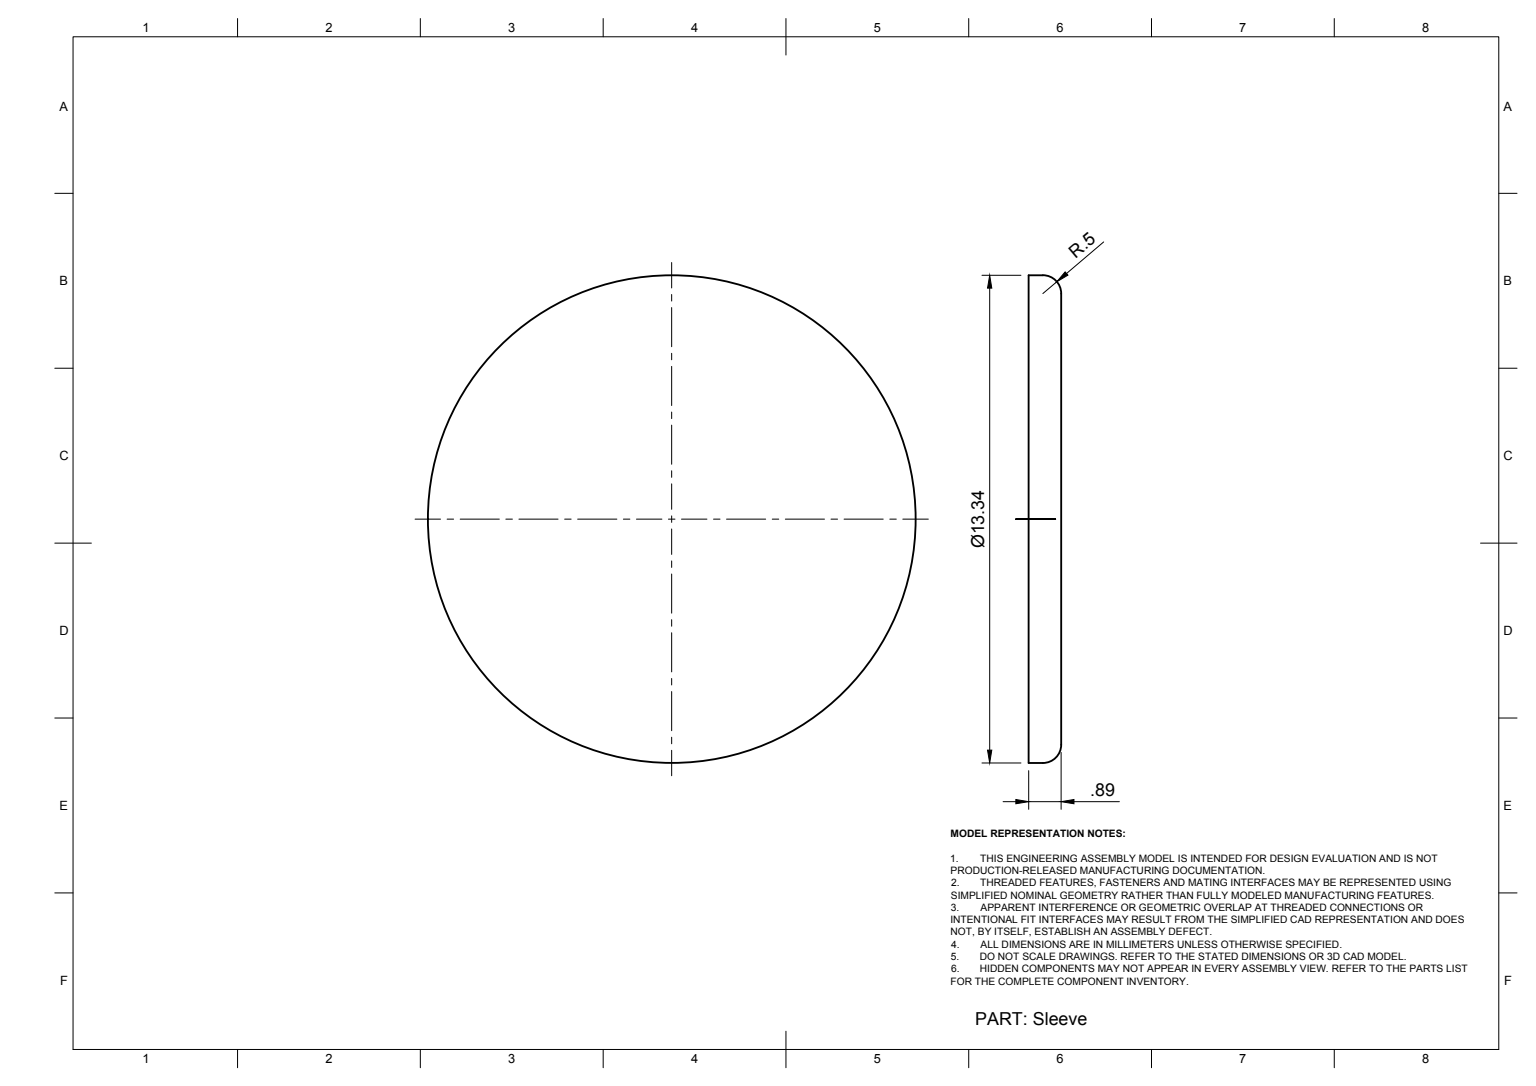
ISO-10303-21;
HEADER;
/* Generated by software containing ST-Developer
 * from STEP Tools, Inc. (www.steptools.com) 
 */

FILE_DESCRIPTION(
/* description */ (''),
/* implementation_level */ '2;1');

FILE_NAME(
/* name */ 'Sleeve.step',
/* time_stamp */ '2026-10-05T01:33:24-07:00',
/* author */ (''),
/* organization */ (''),
/* preprocessor_version */ 'ST-DEVELOPER v20.2',
/* originating_system */ 'Autodesk Translation Framework v15.15.0.0',
/* authorisation */ '');

FILE_SCHEMA (('AUTOMOTIVE_DESIGN { 1 0 10303 214 3 1 1 }'));
ENDSEC;

DATA;
#10=MECHANICAL_DESIGN_GEOMETRIC_PRESENTATION_REPRESENTATION('',(#89),#1128);
#54=TOROIDAL_SURFACE('',#709,6.1693331034204,0.499999999999997);
#69=SHAPE_REPRESENTATION_RELATIONSHIP('SRR','None',#1173,#79);
#79=ADVANCED_BREP_SHAPE_REPRESENTATION('',(#99),#1125);
#89=STYLED_ITEM('',(#1227),#99);
#99=MANIFOLD_SOLID_BREP('Body1',#528);
#114=LINE('',#1064,#131);
#131=VECTOR('',#895,6.66933310342039);
#143=CYLINDRICAL_SURFACE('',#712,6.66933310342039);
#175=FACE_OUTER_BOUND('',#216,.T.);
#176=FACE_OUTER_BOUND('',#217,.T.);
#177=FACE_OUTER_BOUND('',#218,.T.);
#178=FACE_OUTER_BOUND('',#219,.T.);
#216=EDGE_LOOP('',(#426));
#217=EDGE_LOOP('',(#427));
#218=EDGE_LOOP('',(#428,#429,#430,#431));
#219=EDGE_LOOP('',(#432,#433,#434,#435));
#253=CIRCLE('',#706,6.66933310342039);
#254=CIRCLE('',#708,6.16933310342039);
#255=CIRCLE('',#710,6.66933310342039);
#256=CIRCLE('',#711,0.499999999999997);
#287=VERTEX_POINT('',#1054);
#288=VERTEX_POINT('',#1057);
#289=VERTEX_POINT('',#1060);
#335=EDGE_CURVE('',#287,#287,#253,.T.);
#336=EDGE_CURVE('',#288,#288,#254,.T.);
#337=EDGE_CURVE('',#289,#289,#255,.T.);
#338=EDGE_CURVE('',#289,#288,#256,.T.);
#339=EDGE_CURVE('',#287,#289,#114,.T.);
#426=ORIENTED_EDGE('',*,*,#335,.T.);
#427=ORIENTED_EDGE('',*,*,#336,.F.);
#428=ORIENTED_EDGE('',*,*,#337,.F.);
#429=ORIENTED_EDGE('',*,*,#338,.T.);
#430=ORIENTED_EDGE('',*,*,#336,.T.);
#431=ORIENTED_EDGE('',*,*,#338,.F.);
#432=ORIENTED_EDGE('',*,*,#335,.F.);
#433=ORIENTED_EDGE('',*,*,#339,.T.);
#434=ORIENTED_EDGE('',*,*,#337,.T.);
#435=ORIENTED_EDGE('',*,*,#339,.F.);
#474=PLANE('',#705);
#475=PLANE('',#707);
#509=ADVANCED_FACE('',(#175),#474,.T.);
#510=ADVANCED_FACE('',(#176),#475,.T.);
#511=ADVANCED_FACE('',(#177),#54,.T.);
#512=ADVANCED_FACE('',(#178),#143,.T.);
#528=CLOSED_SHELL('',(#509,#510,#511,#512));
#704=AXIS2_PLACEMENT_3D('',#1052,#877,#878);
#705=AXIS2_PLACEMENT_3D('',#1053,#879,#880);
#706=AXIS2_PLACEMENT_3D('',#1055,#881,#882);
#707=AXIS2_PLACEMENT_3D('',#1056,#883,#884);
#708=AXIS2_PLACEMENT_3D('',#1058,#885,#886);
#709=AXIS2_PLACEMENT_3D('',#1059,#887,#888);
#710=AXIS2_PLACEMENT_3D('',#1061,#889,#890);
#711=AXIS2_PLACEMENT_3D('',#1062,#891,#892);
#712=AXIS2_PLACEMENT_3D('',#1063,#893,#894);
#877=DIRECTION('axis',(0.,0.,1.));
#878=DIRECTION('refdir',(1.,0.,0.));
#879=DIRECTION('center_axis',(1.,0.,0.));
#880=DIRECTION('ref_axis',(0.,0.,-1.));
#881=DIRECTION('center_axis',(1.,0.,0.));
#882=DIRECTION('ref_axis',(0.,0.,-1.));
#883=DIRECTION('center_axis',(-1.,0.,0.));
#884=DIRECTION('ref_axis',(0.,0.,1.));
#885=DIRECTION('center_axis',(1.,0.,0.));
#886=DIRECTION('ref_axis',(0.,0.,-1.));
#887=DIRECTION('center_axis',(1.,0.,0.));
#888=DIRECTION('ref_axis',(0.,0.,-1.));
#889=DIRECTION('center_axis',(1.,0.,0.));
#890=DIRECTION('ref_axis',(0.,0.,-1.));
#891=DIRECTION('center_axis',(0.,-1.,-1.22464679914735E-16));
#892=DIRECTION('ref_axis',(0.,-1.22464679914735E-16,1.));
#893=DIRECTION('center_axis',(1.,0.,0.));
#894=DIRECTION('ref_axis',(0.,0.,-1.));
#895=DIRECTION('',(-1.,0.,0.));
#1052=CARTESIAN_POINT('',(0.,0.,0.));
#1053=CARTESIAN_POINT('Origin',(31.9264360344922,0.,0.));
#1054=CARTESIAN_POINT('',(31.9264360344922,-8.16757743755127E-16,6.66933310342039));
#1055=CARTESIAN_POINT('Origin',(31.9264360344922,0.,0.));
#1056=CARTESIAN_POINT('Origin',(31.0379185953459,0.,-6.16933310342039));
#1057=CARTESIAN_POINT('',(31.0379185953459,-7.55525403797759E-16,6.16933310342039));
#1058=CARTESIAN_POINT('Origin',(31.0379185953459,0.,0.));
#1059=CARTESIAN_POINT('Origin',(31.5379185953459,0.,0.));
#1060=CARTESIAN_POINT('',(31.5379185953459,-8.16757743755127E-16,6.66933310342039));
#1061=CARTESIAN_POINT('Origin',(31.5379185953459,0.,0.));
#1062=CARTESIAN_POINT('Origin',(31.5379185953459,-7.5552540379776E-16,6.1693331034204));
#1063=CARTESIAN_POINT('Origin',(31.7321773149191,0.,0.));
#1064=CARTESIAN_POINT('',(31.7321773149191,-8.16757743755127E-16,6.66933310342039));
#1113=UNCERTAINTY_MEASURE_WITH_UNIT(LENGTH_MEASURE(0.01),#1129,
'DISTANCE_ACCURACY_VALUE',
'Maximum model space distance between geometric entities at asserted c
onnectivities');
#1116=UNCERTAINTY_MEASURE_WITH_UNIT(LENGTH_MEASURE(0.01),#1129,
'DISTANCE_ACCURACY_VALUE',
'Maximum model space distance between geometric entities at asserted c
onnectivities');
#1125=(
GEOMETRIC_REPRESENTATION_CONTEXT(3)
GLOBAL_UNCERTAINTY_ASSIGNED_CONTEXT((#1113))
GLOBAL_UNIT_ASSIGNED_CONTEXT((#1129,#1131,#1132))
REPRESENTATION_CONTEXT('','3D')
);
#1128=(
GEOMETRIC_REPRESENTATION_CONTEXT(3)
GLOBAL_UNCERTAINTY_ASSIGNED_CONTEXT((#1116))
GLOBAL_UNIT_ASSIGNED_CONTEXT((#1129,#1131,#1132))
REPRESENTATION_CONTEXT('','3D')
);
#1129=(
LENGTH_UNIT()
NAMED_UNIT(*)
SI_UNIT(.MILLI.,.METRE.)
);
#1131=(
NAMED_UNIT(*)
PLANE_ANGLE_UNIT()
SI_UNIT($,.RADIAN.)
);
#1132=(
NAMED_UNIT(*)
SI_UNIT($,.STERADIAN.)
SOLID_ANGLE_UNIT()
);
#1141=SHAPE_DEFINITION_REPRESENTATION(#1152,#1173);
#1152=PRODUCT_DEFINITION_SHAPE('',$,#1185);
#1173=SHAPE_REPRESENTATION('',(#704),#1125);
#1176=PRODUCT_DEFINITION_CONTEXT('part definition',#1211,'design');
#1185=PRODUCT_DEFINITION('Sleeve','Sleeve',#1196,#1176);
#1196=PRODUCT_DEFINITION_FORMATION('',$,#1221);
#1211=APPLICATION_CONTEXT(
'Core Data for Automotive Mechanical Design Process');
#1212=PRODUCT_CONTEXT('part definition',#1211,'mechanical');
#1221=PRODUCT('Sleeve','Sleeve',$,(#1212));
#1227=PRESENTATION_STYLE_ASSIGNMENT((#1231));
#1231=SURFACE_STYLE_USAGE(.BOTH.,#1235);
#1235=SURFACE_SIDE_STYLE('',(#1239));
#1239=SURFACE_STYLE_FILL_AREA(#1243);
#1243=FILL_AREA_STYLE('Opaque(77,77,77)',(#1247));
#1247=FILL_AREA_STYLE_COLOUR('Opaque(77,77,77)',#1251);
#1251=COLOUR_RGB('Opaque(77,77,77)', 0.72549020, 0.75294118, 0.79215686);
ENDSEC;
END-ISO-10303-21;
